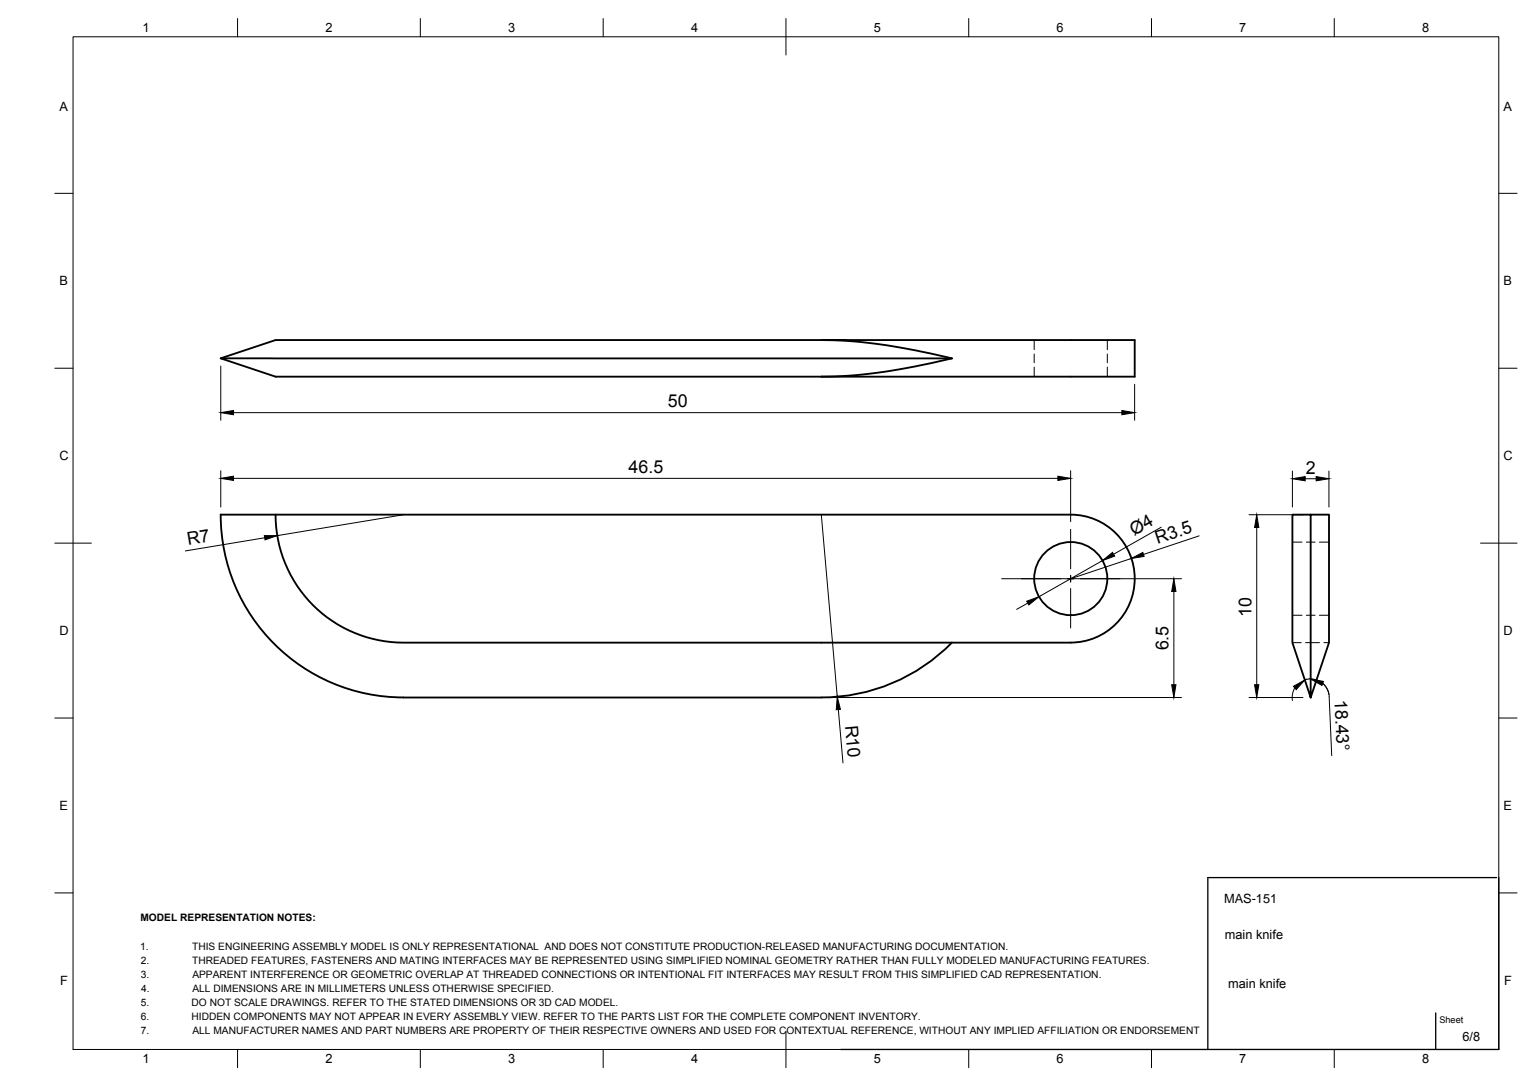
ISO-10303-21;
HEADER;
/* Generated by software containing ST-Developer
 * from STEP Tools, Inc. (www.steptools.com) 
 */

FILE_DESCRIPTION(
/* description */ ('STEP AP214'),
/* implementation_level */ '2;1');

FILE_NAME(
/* name */ 'main knife.step',
/* time_stamp */ '2026-11-04T19:14:12-08:00',
/* author */ (''),
/* organization */ (''),
/* preprocessor_version */ 'ST-DEVELOPER v20.2',
/* originating_system */ 'Autodesk Translation Framework v15.17.0.0',
/* authorisation */ '');

FILE_SCHEMA (('AUTOMOTIVE_DESIGN { 1 0 10303 214 3 1 1 }'));
ENDSEC;

DATA;
#10=MECHANICAL_DESIGN_GEOMETRIC_PRESENTATION_REPRESENTATION('',(#101),#5990);
#73=CONICAL_SURFACE('',#3531,6.99999999999997,1.24904577239826);
#74=CONICAL_SURFACE('',#3534,6.99999999999997,1.24904577239826);
#75=CONICAL_SURFACE('',#3535,6.99999999999997,1.24904577239826);
#76=CONICAL_SURFACE('',#3538,6.99999999999997,1.24904577239826);
#81=(
BOUNDED_CURVE()
B_SPLINE_CURVE(2,(#5211,#5212,#5213),.UNSPECIFIED.,.F.,.F.)
B_SPLINE_CURVE_WITH_KNOTS((3,3),(1.46969384566992,2.45666783066589),
 .UNSPECIFIED.)
CURVE()
GEOMETRIC_REPRESENTATION_ITEM()
RATIONAL_B_SPLINE_CURVE((1.64285714285714,1.64285714285714,1.35294117647059))
REPRESENTATION_ITEM('')
);
#82=(
BOUNDED_CURVE()
B_SPLINE_CURVE(2,(#5214,#5215,#5216),.UNSPECIFIED.,.F.,.F.)
B_SPLINE_CURVE_WITH_KNOTS((3,3),(0.482719860673933,1.46969384566992),
 .UNSPECIFIED.)
CURVE()
GEOMETRIC_REPRESENTATION_ITEM()
RATIONAL_B_SPLINE_CURVE((1.35294117647058,1.64285714285714,1.64285714285714))
REPRESENTATION_ITEM('')
);
#87=SHAPE_REPRESENTATION_RELATIONSHIP('SRR','None',#6023,#94);
#94=ADVANCED_BREP_SHAPE_REPRESENTATION('',(#108),#5985);
#101=STYLED_ITEM('',(#6066),#108);
#108=MANIFOLD_SOLID_BREP('Body1',#3271);
#127=FACE_BOUND('',#534,.T.);
#128=FACE_BOUND('',#536,.T.);
#200=PLANE('',#3523);
#201=PLANE('',#3524);
#202=PLANE('',#3525);
#203=PLANE('',#3528);
#204=PLANE('',#3533);
#205=PLANE('',#3537);
#338=FACE_OUTER_BOUND('',#530,.T.);
#339=FACE_OUTER_BOUND('',#531,.T.);
#340=FACE_OUTER_BOUND('',#532,.T.);
#341=FACE_OUTER_BOUND('',#533,.T.);
#342=FACE_OUTER_BOUND('',#535,.T.);
#343=FACE_OUTER_BOUND('',#537,.T.);
#344=FACE_OUTER_BOUND('',#538,.T.);
#345=FACE_OUTER_BOUND('',#539,.T.);
#346=FACE_OUTER_BOUND('',#540,.T.);
#347=FACE_OUTER_BOUND('',#541,.T.);
#348=FACE_OUTER_BOUND('',#542,.T.);
#349=FACE_OUTER_BOUND('',#543,.T.);
#530=EDGE_LOOP('',(#2650,#2651,#2652,#2653));
#531=EDGE_LOOP('',(#2654,#2655,#2656,#2657,#2658));
#532=EDGE_LOOP('',(#2659,#2660,#2661,#2662,#2663));
#533=EDGE_LOOP('',(#2664,#2665,#2666,#2667,#2668));
#534=EDGE_LOOP('',(#2669));
#535=EDGE_LOOP('',(#2670,#2671,#2672,#2673,#2674));
#536=EDGE_LOOP('',(#2675));
#537=EDGE_LOOP('',(#2676,#2677,#2678));
#538=EDGE_LOOP('',(#2679,#2680,#2681,#2682));
#539=EDGE_LOOP('',(#2683,#2684,#2685));
#540=EDGE_LOOP('',(#2686,#2687,#2688,#2689));
#541=EDGE_LOOP('',(#2690,#2691,#2692,#2693));
#542=EDGE_LOOP('',(#2694,#2695,#2696,#2697));
#543=EDGE_LOOP('',(#2698,#2699,#2700,#2701));
#826=LINE('',#5200,#1129);
#827=LINE('',#5205,#1130);
#828=LINE('',#5207,#1131);
#829=LINE('',#5209,#1132);
#830=LINE('',#5220,#1133);
#831=LINE('',#5222,#1134);
#832=LINE('',#5224,#1135);
#833=LINE('',#5226,#1136);
#834=LINE('',#5227,#1137);
#835=LINE('',#5231,#1138);
#836=LINE('',#5237,#1139);
#837=LINE('',#5241,#1140);
#838=LINE('',#5244,#1141);
#839=LINE('',#5245,#1142);
#840=LINE('',#5247,#1143);
#841=LINE('',#5251,#1144);
#1129=VECTOR('',#4225,2.);
#1130=VECTOR('',#4230,1000.);
#1131=VECTOR('',#4231,1000.);
#1132=VECTOR('',#4232,1000.);
#1133=VECTOR('',#4235,1000.);
#1134=VECTOR('',#4236,1000.);
#1135=VECTOR('',#4237,1000.);
#1136=VECTOR('',#4238,1000.);
#1137=VECTOR('',#4239,1000.);
#1138=VECTOR('',#4244,1000.);
#1139=VECTOR('',#4253,1000.);
#1140=VECTOR('',#4258,1000.);
#1141=VECTOR('',#4261,1000.);
#1142=VECTOR('',#4262,1000.);
#1143=VECTOR('',#4265,1000.);
#1144=VECTOR('',#4272,1000.);
#1294=CIRCLE('',#3521,2.);
#1295=CIRCLE('',#3522,2.);
#1296=CIRCLE('',#3526,3.5);
#1297=CIRCLE('',#3527,6.99999999999997);
#1298=CIRCLE('',#3529,3.5);
#1299=CIRCLE('',#3530,6.99999999999997);
#1300=CIRCLE('',#3532,10.);
#1301=CIRCLE('',#3536,10.);
#1532=VERTEX_POINT('',#5197);
#1533=VERTEX_POINT('',#5199);
#1534=VERTEX_POINT('',#5203);
#1535=VERTEX_POINT('',#5204);
#1536=VERTEX_POINT('',#5206);
#1537=VERTEX_POINT('',#5208);
#1538=VERTEX_POINT('',#5210);
#1539=VERTEX_POINT('',#5218);
#1540=VERTEX_POINT('',#5219);
#1541=VERTEX_POINT('',#5221);
#1542=VERTEX_POINT('',#5223);
#1543=VERTEX_POINT('',#5225);
#1544=VERTEX_POINT('',#5230);
#1545=VERTEX_POINT('',#5235);
#1546=VERTEX_POINT('',#5239);
#1547=VERTEX_POINT('',#5243);
#1921=EDGE_CURVE('',#1532,#1532,#1294,.T.);
#1922=EDGE_CURVE('',#1532,#1533,#826,.T.);
#1923=EDGE_CURVE('',#1533,#1533,#1295,.T.);
#1924=EDGE_CURVE('',#1534,#1535,#827,.T.);
#1925=EDGE_CURVE('',#1534,#1536,#828,.T.);
#1926=EDGE_CURVE('',#1536,#1537,#829,.T.);
#1927=EDGE_CURVE('',#1537,#1538,#81,.T.);
#1928=EDGE_CURVE('',#1538,#1535,#82,.T.);
#1929=EDGE_CURVE('',#1539,#1540,#830,.T.);
#1930=EDGE_CURVE('',#1539,#1541,#831,.T.);
#1931=EDGE_CURVE('',#1541,#1542,#832,.T.);
#1932=EDGE_CURVE('',#1542,#1543,#833,.T.);
#1933=EDGE_CURVE('',#1543,#1540,#834,.T.);
#1934=EDGE_CURVE('',#1541,#1534,#1296,.T.);
#1935=EDGE_CURVE('',#1535,#1544,#835,.T.);
#1936=EDGE_CURVE('',#1544,#1542,#1297,.T.);
#1937=EDGE_CURVE('',#1536,#1539,#1298,.T.);
#1938=EDGE_CURVE('',#1540,#1545,#1299,.T.);
#1939=EDGE_CURVE('',#1545,#1537,#836,.T.);
#1940=EDGE_CURVE('',#1538,#1546,#1300,.T.);
#1941=EDGE_CURVE('',#1546,#1537,#837,.T.);
#1942=EDGE_CURVE('',#1547,#1545,#838,.T.);
#1943=EDGE_CURVE('',#1546,#1547,#839,.T.);
#1944=EDGE_CURVE('',#1535,#1546,#840,.T.);
#1945=EDGE_CURVE('',#1547,#1543,#1301,.T.);
#1946=EDGE_CURVE('',#1544,#1547,#841,.T.);
#2650=ORIENTED_EDGE('',*,*,#1921,.F.);
#2651=ORIENTED_EDGE('',*,*,#1922,.T.);
#2652=ORIENTED_EDGE('',*,*,#1923,.T.);
#2653=ORIENTED_EDGE('',*,*,#1922,.F.);
#2654=ORIENTED_EDGE('',*,*,#1924,.F.);
#2655=ORIENTED_EDGE('',*,*,#1925,.T.);
#2656=ORIENTED_EDGE('',*,*,#1926,.T.);
#2657=ORIENTED_EDGE('',*,*,#1927,.T.);
#2658=ORIENTED_EDGE('',*,*,#1928,.T.);
#2659=ORIENTED_EDGE('',*,*,#1929,.F.);
#2660=ORIENTED_EDGE('',*,*,#1930,.T.);
#2661=ORIENTED_EDGE('',*,*,#1931,.T.);
#2662=ORIENTED_EDGE('',*,*,#1932,.T.);
#2663=ORIENTED_EDGE('',*,*,#1933,.T.);
#2664=ORIENTED_EDGE('',*,*,#1931,.F.);
#2665=ORIENTED_EDGE('',*,*,#1934,.T.);
#2666=ORIENTED_EDGE('',*,*,#1924,.T.);
#2667=ORIENTED_EDGE('',*,*,#1935,.T.);
#2668=ORIENTED_EDGE('',*,*,#1936,.T.);
#2669=ORIENTED_EDGE('',*,*,#1923,.F.);
#2670=ORIENTED_EDGE('',*,*,#1937,.T.);
#2671=ORIENTED_EDGE('',*,*,#1929,.T.);
#2672=ORIENTED_EDGE('',*,*,#1938,.T.);
#2673=ORIENTED_EDGE('',*,*,#1939,.T.);
#2674=ORIENTED_EDGE('',*,*,#1926,.F.);
#2675=ORIENTED_EDGE('',*,*,#1921,.T.);
#2676=ORIENTED_EDGE('',*,*,#1940,.F.);
#2677=ORIENTED_EDGE('',*,*,#1927,.F.);
#2678=ORIENTED_EDGE('',*,*,#1941,.F.);
#2679=ORIENTED_EDGE('',*,*,#1941,.T.);
#2680=ORIENTED_EDGE('',*,*,#1939,.F.);
#2681=ORIENTED_EDGE('',*,*,#1942,.F.);
#2682=ORIENTED_EDGE('',*,*,#1943,.F.);
#2683=ORIENTED_EDGE('',*,*,#1928,.F.);
#2684=ORIENTED_EDGE('',*,*,#1940,.T.);
#2685=ORIENTED_EDGE('',*,*,#1944,.F.);
#2686=ORIENTED_EDGE('',*,*,#1938,.F.);
#2687=ORIENTED_EDGE('',*,*,#1933,.F.);
#2688=ORIENTED_EDGE('',*,*,#1945,.F.);
#2689=ORIENTED_EDGE('',*,*,#1942,.T.);
#2690=ORIENTED_EDGE('',*,*,#1944,.T.);
#2691=ORIENTED_EDGE('',*,*,#1943,.T.);
#2692=ORIENTED_EDGE('',*,*,#1946,.F.);
#2693=ORIENTED_EDGE('',*,*,#1935,.F.);
#2694=ORIENTED_EDGE('',*,*,#1946,.T.);
#2695=ORIENTED_EDGE('',*,*,#1945,.T.);
#2696=ORIENTED_EDGE('',*,*,#1932,.F.);
#2697=ORIENTED_EDGE('',*,*,#1936,.F.);
#2698=ORIENTED_EDGE('',*,*,#1925,.F.);
#2699=ORIENTED_EDGE('',*,*,#1934,.F.);
#2700=ORIENTED_EDGE('',*,*,#1930,.F.);
#2701=ORIENTED_EDGE('',*,*,#1937,.F.);
#3061=CYLINDRICAL_SURFACE('',#3520,2.);
#3062=CYLINDRICAL_SURFACE('',#3539,3.5);
#3187=ADVANCED_FACE('',(#338),#3061,.F.);
#3188=ADVANCED_FACE('',(#339),#200,.F.);
#3189=ADVANCED_FACE('',(#340),#201,.T.);
#3190=ADVANCED_FACE('',(#341,#127),#202,.T.);
#3191=ADVANCED_FACE('',(#342,#128),#203,.F.);
#3192=ADVANCED_FACE('',(#343),#73,.T.);
#3193=ADVANCED_FACE('',(#344),#204,.T.);
#3194=ADVANCED_FACE('',(#345),#74,.T.);
#3195=ADVANCED_FACE('',(#346),#75,.T.);
#3196=ADVANCED_FACE('',(#347),#205,.F.);
#3197=ADVANCED_FACE('',(#348),#76,.T.);
#3198=ADVANCED_FACE('',(#349),#3062,.T.);
#3271=CLOSED_SHELL('',(#3187,#3188,#3189,#3190,#3191,#3192,#3193,#3194,
#3195,#3196,#3197,#3198));
#3519=AXIS2_PLACEMENT_3D('',#5195,#4219,#4220);
#3520=AXIS2_PLACEMENT_3D('',#5196,#4221,#4222);
#3521=AXIS2_PLACEMENT_3D('',#5198,#4223,#4224);
#3522=AXIS2_PLACEMENT_3D('',#5201,#4226,#4227);
#3523=AXIS2_PLACEMENT_3D('',#5202,#4228,#4229);
#3524=AXIS2_PLACEMENT_3D('',#5217,#4233,#4234);
#3525=AXIS2_PLACEMENT_3D('',#5228,#4240,#4241);
#3526=AXIS2_PLACEMENT_3D('',#5229,#4242,#4243);
#3527=AXIS2_PLACEMENT_3D('',#5232,#4245,#4246);
#3528=AXIS2_PLACEMENT_3D('',#5233,#4247,#4248);
#3529=AXIS2_PLACEMENT_3D('',#5234,#4249,#4250);
#3530=AXIS2_PLACEMENT_3D('',#5236,#4251,#4252);
#3531=AXIS2_PLACEMENT_3D('',#5238,#4254,#4255);
#3532=AXIS2_PLACEMENT_3D('',#5240,#4256,#4257);
#3533=AXIS2_PLACEMENT_3D('',#5242,#4259,#4260);
#3534=AXIS2_PLACEMENT_3D('',#5246,#4263,#4264);
#3535=AXIS2_PLACEMENT_3D('',#5248,#4266,#4267);
#3536=AXIS2_PLACEMENT_3D('',#5249,#4268,#4269);
#3537=AXIS2_PLACEMENT_3D('',#5250,#4270,#4271);
#3538=AXIS2_PLACEMENT_3D('',#5252,#4273,#4274);
#3539=AXIS2_PLACEMENT_3D('',#5253,#4275,#4276);
#4219=DIRECTION('axis',(0.,0.,1.));
#4220=DIRECTION('refdir',(1.,0.,0.));
#4221=DIRECTION('center_axis',(0.,0.,-1.));
#4222=DIRECTION('ref_axis',(-1.,0.,0.));
#4223=DIRECTION('center_axis',(0.,0.,-1.));
#4224=DIRECTION('ref_axis',(-1.,0.,0.));
#4225=DIRECTION('',(0.,0.,-1.));
#4226=DIRECTION('center_axis',(0.,0.,-1.));
#4227=DIRECTION('ref_axis',(-1.,0.,0.));
#4228=DIRECTION('center_axis',(1.,0.,0.));
#4229=DIRECTION('ref_axis',(0.,0.,-1.));
#4230=DIRECTION('',(0.,1.,0.));
#4231=DIRECTION('',(0.,0.,1.));
#4232=DIRECTION('',(0.,1.,0.));
#4233=DIRECTION('center_axis',(1.,0.,0.));
#4234=DIRECTION('ref_axis',(0.,0.,-1.));
#4235=DIRECTION('',(0.,1.,0.));
#4236=DIRECTION('',(0.,0.,-1.));
#4237=DIRECTION('',(0.,1.,0.));
#4238=DIRECTION('',(0.,0.948683298050515,0.316227766016835));
#4239=DIRECTION('',(0.,-0.948683298050515,0.316227766016835));
#4240=DIRECTION('center_axis',(0.,0.,-1.));
#4241=DIRECTION('ref_axis',(-1.,0.,0.));
#4242=DIRECTION('center_axis',(0.,0.,-1.));
#4243=DIRECTION('ref_axis',(-1.,0.,0.));
#4244=DIRECTION('',(0.,1.,0.));
#4245=DIRECTION('center_axis',(0.,0.,-1.));
#4246=DIRECTION('ref_axis',(-1.,0.,0.));
#4247=DIRECTION('center_axis',(0.,0.,-1.));
#4248=DIRECTION('ref_axis',(-1.,0.,0.));
#4249=DIRECTION('center_axis',(0.,0.,1.));
#4250=DIRECTION('ref_axis',(-1.,0.,0.));
#4251=DIRECTION('center_axis',(0.,0.,1.));
#4252=DIRECTION('ref_axis',(-1.,0.,0.));
#4253=DIRECTION('',(0.,-1.,0.));
#4254=DIRECTION('center_axis',(0.,0.,-1.));
#4255=DIRECTION('ref_axis',(-1.,0.,0.));
#4256=DIRECTION('center_axis',(0.,0.,-1.));
#4257=DIRECTION('ref_axis',(-1.,0.,0.));
#4258=DIRECTION('',(0.948683298050515,0.,0.316227766016835));
#4259=DIRECTION('center_axis',(-0.316227766016835,0.,0.948683298050515));
#4260=DIRECTION('ref_axis',(0.,-1.,0.));
#4261=DIRECTION('',(0.948683298050515,0.,0.316227766016835));
#4262=DIRECTION('',(0.,1.,0.));
#4263=DIRECTION('center_axis',(0.,0.,1.));
#4264=DIRECTION('ref_axis',(1.,0.,0.));
#4265=DIRECTION('',(-0.948683298050515,0.,0.316227766016835));
#4266=DIRECTION('center_axis',(0.,0.,-1.));
#4267=DIRECTION('ref_axis',(-1.,0.,0.));
#4268=DIRECTION('center_axis',(0.,0.,-1.));
#4269=DIRECTION('ref_axis',(-1.,0.,0.));
#4270=DIRECTION('center_axis',(0.316227766016835,0.,0.948683298050515));
#4271=DIRECTION('ref_axis',(0.,-1.,0.));
#4272=DIRECTION('',(-0.948683298050515,0.,0.316227766016835));
#4273=DIRECTION('center_axis',(0.,0.,1.));
#4274=DIRECTION('ref_axis',(1.,0.,0.));
#4275=DIRECTION('center_axis',(0.,0.,1.));
#4276=DIRECTION('ref_axis',(1.,0.,0.));
#5195=CARTESIAN_POINT('',(0.,0.,0.));
#5196=CARTESIAN_POINT('Origin',(-16.,-116.5,6.07153216591882E-15));
#5197=CARTESIAN_POINT('',(-14.,-116.5,6.07153216591882E-15));
#5198=CARTESIAN_POINT('Origin',(-16.,-116.5,6.07153216591882E-15));
#5199=CARTESIAN_POINT('',(-14.,-116.5,-2.));
#5200=CARTESIAN_POINT('',(-14.,-116.5,6.07153216591882E-15));
#5201=CARTESIAN_POINT('Origin',(-16.,-116.5,-2.));
#5202=CARTESIAN_POINT('Origin',(-19.5,-120.,-2.));
#5203=CARTESIAN_POINT('',(-19.5,-116.5,-2.));
#5204=CARTESIAN_POINT('',(-19.5,-102.858571571457,-2.));
#5205=CARTESIAN_POINT('',(-19.5,-120.,-2.));
#5206=CARTESIAN_POINT('',(-19.5,-116.5,0.));
#5207=CARTESIAN_POINT('',(-19.5,-116.5,-2.));
#5208=CARTESIAN_POINT('',(-19.5,-102.858571571457,0.));
#5209=CARTESIAN_POINT('',(-19.5,-120.,0.));
#5210=CARTESIAN_POINT('',(-19.5,-110.,-0.999999999999999));
#5211=CARTESIAN_POINT('Ctrl Pts',(-19.5,-102.858571571457,-1.05422916773102E-14));
#5212=CARTESIAN_POINT('Ctrl Pts',(-19.5,-105.799159747916,-1.69574446668887E-14));
#5213=CARTESIAN_POINT('Ctrl Pts',(-19.5,-110.,-1.));
#5214=CARTESIAN_POINT('Ctrl Pts',(-19.5,-110.,-0.999999999999976));
#5215=CARTESIAN_POINT('Ctrl Pts',(-19.5,-105.799159747916,-1.99999999999999));
#5216=CARTESIAN_POINT('Ctrl Pts',(-19.5,-102.858571571457,-1.99999999999999));
#5217=CARTESIAN_POINT('Origin',(-12.5,-120.,-2.));
#5218=CARTESIAN_POINT('',(-12.5,-116.5,0.));
#5219=CARTESIAN_POINT('',(-12.5,-73.0000000000001,0.));
#5220=CARTESIAN_POINT('',(-12.5,-120.,0.));
#5221=CARTESIAN_POINT('',(-12.5,-116.5,-2.));
#5222=CARTESIAN_POINT('',(-12.5,-116.5,-2.));
#5223=CARTESIAN_POINT('',(-12.5,-73.0000000000001,-2.));
#5224=CARTESIAN_POINT('',(-12.5,-120.,-2.));
#5225=CARTESIAN_POINT('',(-12.5,-70.,-1.));
#5226=CARTESIAN_POINT('',(-12.5,-80.,-4.3333333333333));
#5227=CARTESIAN_POINT('',(-12.5,-80.,2.3333333333333));
#5228=CARTESIAN_POINT('Origin',(0.,0.,-2.));
#5229=CARTESIAN_POINT('Origin',(-16.,-116.5,-2.));
#5230=CARTESIAN_POINT('',(-19.5,-80.,-2.));
#5231=CARTESIAN_POINT('',(-19.5,0.,-2.));
#5232=CARTESIAN_POINT('Origin',(-12.5,-80.,-2.));
#5233=CARTESIAN_POINT('Origin',(0.,0.,0.));
#5234=CARTESIAN_POINT('Origin',(-16.,-116.5,0.));
#5235=CARTESIAN_POINT('',(-19.5,-80.,0.));
#5236=CARTESIAN_POINT('Origin',(-12.5,-80.,0.));
#5237=CARTESIAN_POINT('',(-19.5,-102.858571571457,0.));
#5238=CARTESIAN_POINT('Origin',(-12.5,-102.858571571457,0.));
#5239=CARTESIAN_POINT('',(-22.5,-102.858571571457,-0.999999999999999));
#5240=CARTESIAN_POINT('Origin',(-12.5,-102.858571571457,-1.));
#5241=CARTESIAN_POINT('',(-22.5,-102.858571571457,-1.));
#5242=CARTESIAN_POINT('Origin',(-22.5,0.,-1.));
#5243=CARTESIAN_POINT('',(-22.5,-80.,-0.999999999999999));
#5244=CARTESIAN_POINT('',(-22.5,-80.,-1.));
#5245=CARTESIAN_POINT('',(-22.5,-80.,-1.));
#5246=CARTESIAN_POINT('Origin',(-12.5,-102.858571571457,-2.));
#5247=CARTESIAN_POINT('',(-19.5,-102.858571571457,-2.));
#5248=CARTESIAN_POINT('Origin',(-12.5,-80.,0.));
#5249=CARTESIAN_POINT('Origin',(-12.5,-80.,-1.));
#5250=CARTESIAN_POINT('Origin',(-22.5,0.,-0.999999999999999));
#5251=CARTESIAN_POINT('',(-19.5,-80.,-2.));
#5252=CARTESIAN_POINT('Origin',(-12.5,-80.,-2.));
#5253=CARTESIAN_POINT('Origin',(-16.,-116.5,-2.));
#5976=UNCERTAINTY_MEASURE_WITH_UNIT(LENGTH_MEASURE(0.01),#5991,
'DISTANCE_ACCURACY_VALUE',
'Maximum model space distance between geometric entities at asserted c
onnectivities');
#5981=UNCERTAINTY_MEASURE_WITH_UNIT(LENGTH_MEASURE(0.01),#5991,
'DISTANCE_ACCURACY_VALUE',
'Maximum model space distance between geometric entities at asserted c
onnectivities');
#5985=(
GEOMETRIC_REPRESENTATION_CONTEXT(3)
GLOBAL_UNCERTAINTY_ASSIGNED_CONTEXT((#5976))
GLOBAL_UNIT_ASSIGNED_CONTEXT((#5991,#5993,#5994))
REPRESENTATION_CONTEXT('','3D')
);
#5990=(
GEOMETRIC_REPRESENTATION_CONTEXT(3)
GLOBAL_UNCERTAINTY_ASSIGNED_CONTEXT((#5981))
GLOBAL_UNIT_ASSIGNED_CONTEXT((#5991,#5993,#5994))
REPRESENTATION_CONTEXT('','3D')
);
#5991=(
LENGTH_UNIT()
NAMED_UNIT(*)
SI_UNIT(.MILLI.,.METRE.)
);
#5993=(
NAMED_UNIT(*)
PLANE_ANGLE_UNIT()
SI_UNIT($,.RADIAN.)
);
#5994=(
NAMED_UNIT(*)
SI_UNIT($,.STERADIAN.)
SOLID_ANGLE_UNIT()
);
#5998=SHAPE_DEFINITION_REPRESENTATION(#6006,#6023);
#6006=PRODUCT_DEFINITION_SHAPE('',$,#6032);
#6023=SHAPE_REPRESENTATION('',(#3519),#5985);
#6028=PRODUCT_DEFINITION_CONTEXT('part definition',#6054,'design');
#6032=PRODUCT_DEFINITION('main knife','main knife',#6040,#6028);
#6040=PRODUCT_DEFINITION_FORMATION('',$,#6059);
#6054=APPLICATION_CONTEXT(
'Core Data for Automotive Mechanical Design Process');
#6055=PRODUCT_CONTEXT('part definition',#6054,'mechanical');
#6059=PRODUCT('main knife','main knife',$,(#6055));
#6066=PRESENTATION_STYLE_ASSIGNMENT((#6072));
#6072=SURFACE_STYLE_USAGE(.BOTH.,#6078);
#6078=SURFACE_SIDE_STYLE('',(#6084));
#6084=SURFACE_STYLE_FILL_AREA(#6090);
#6090=FILL_AREA_STYLE('Opaque(97,158,199)',(#6096));
#6096=FILL_AREA_STYLE_COLOUR('Opaque(97,158,199)',#6102);
#6102=COLOUR_RGB('Opaque(97,158,199)',0.380392156862745,0.619607843137255,
0.780392156862745);
ENDSEC;
END-ISO-10303-21;
